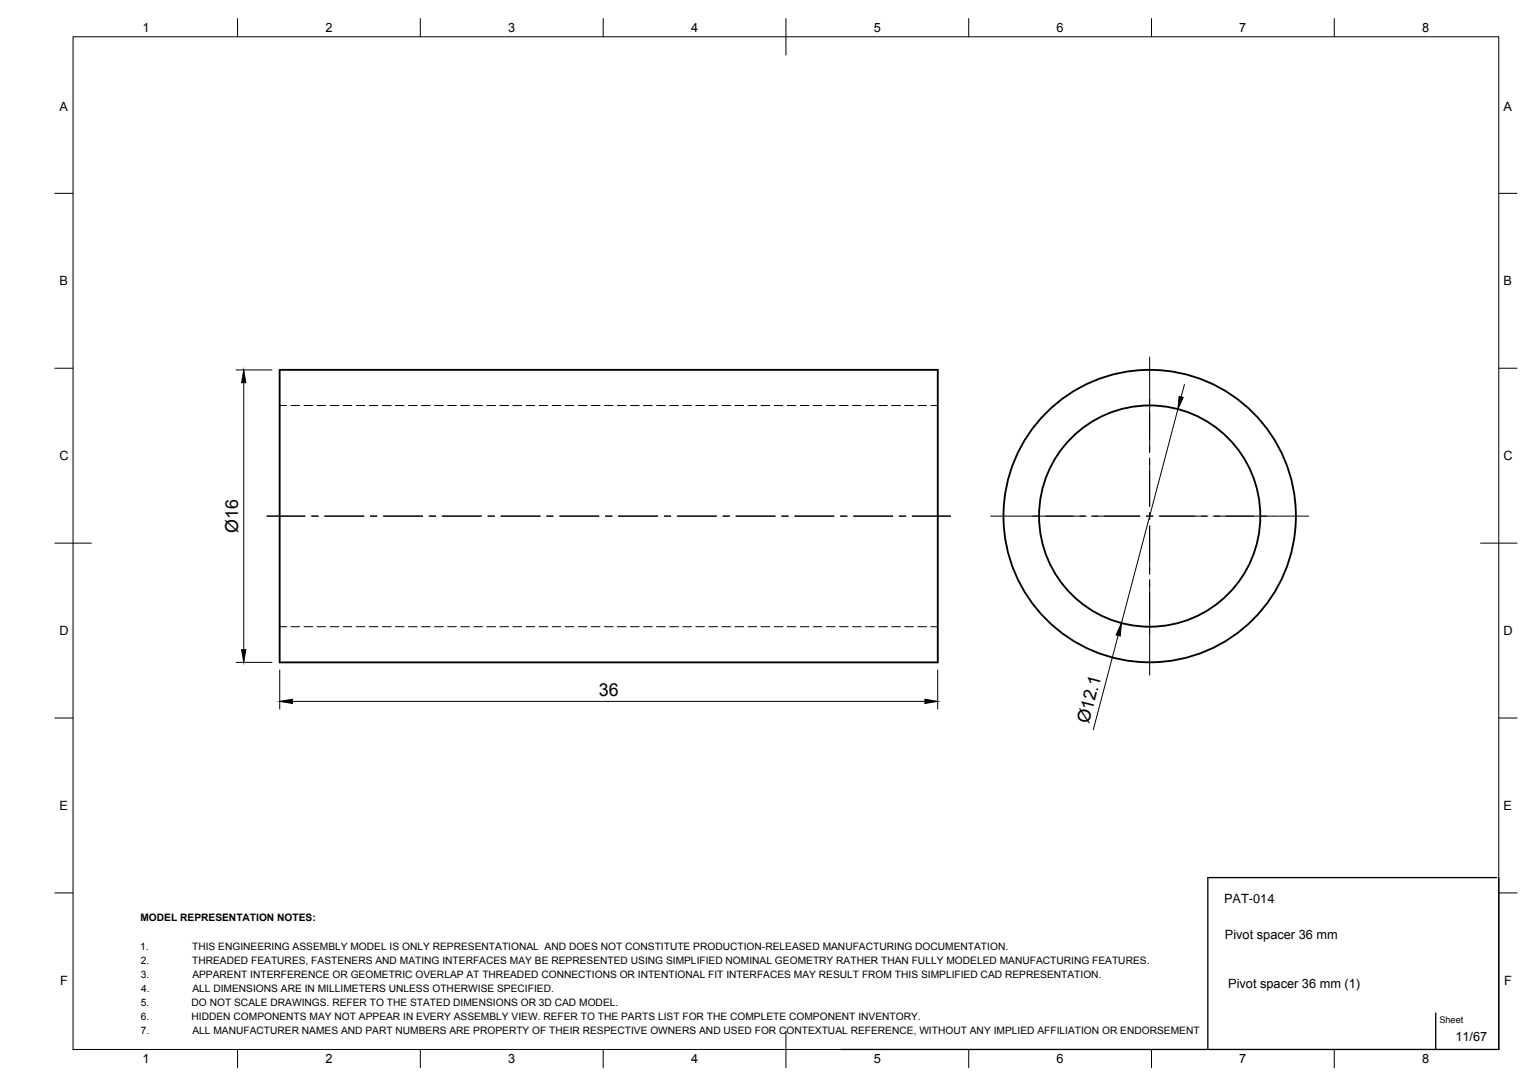
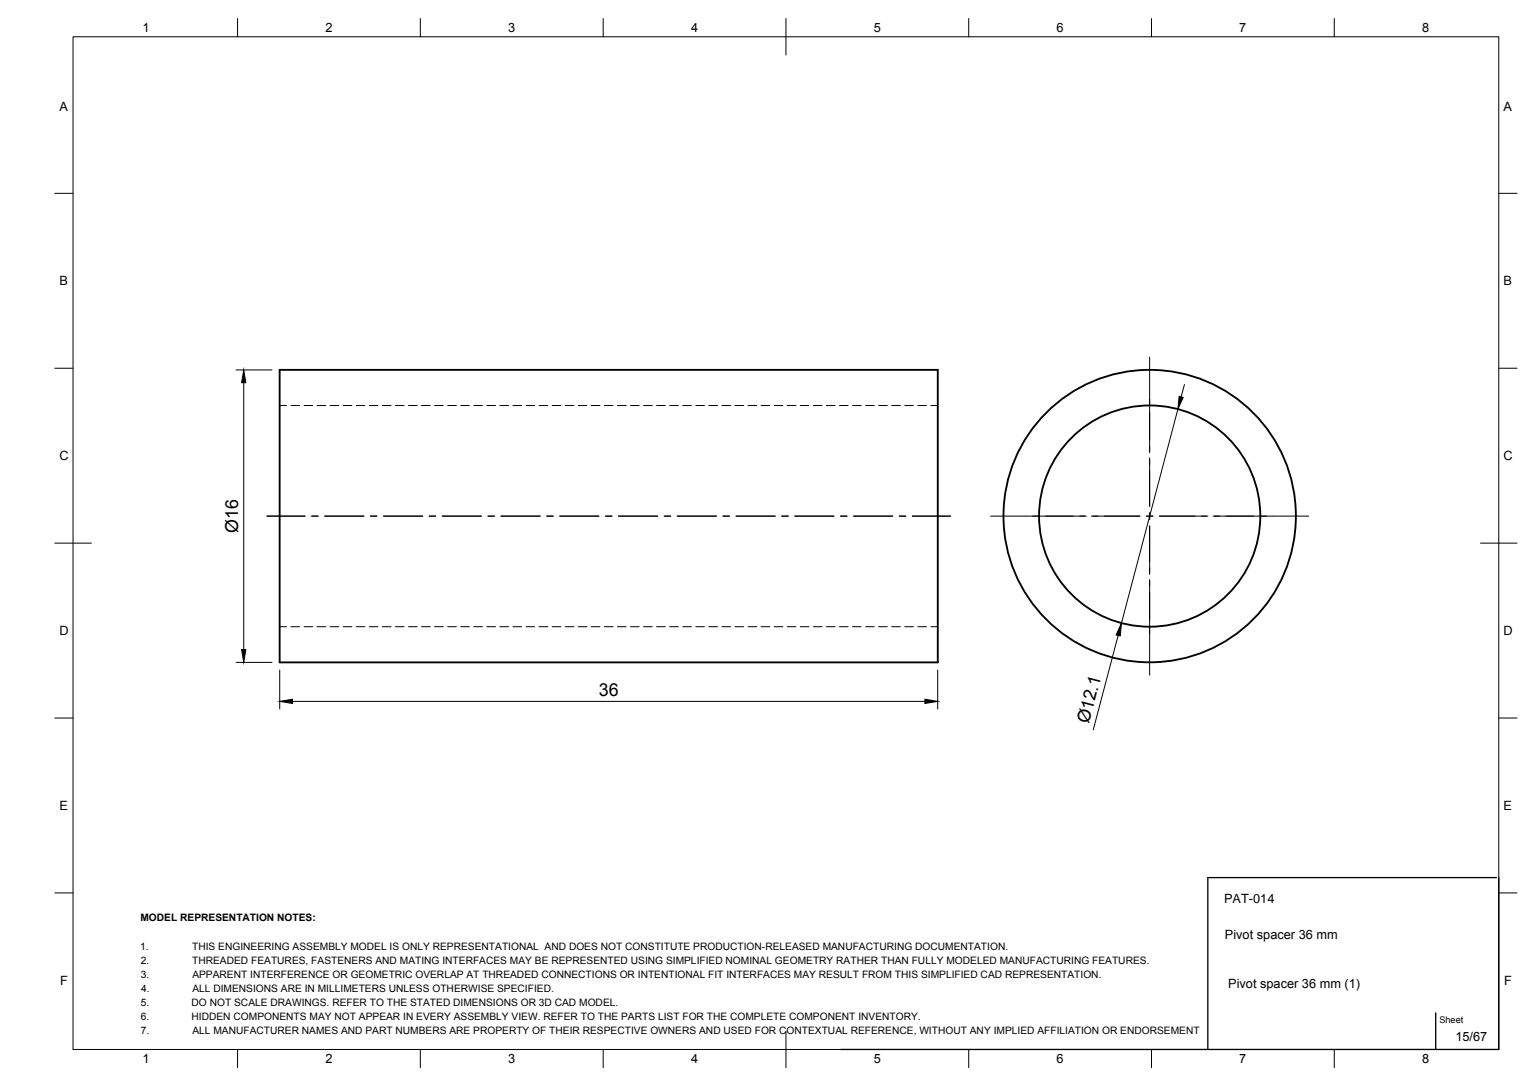
ISO-10303-21;
HEADER;
/* Generated by software containing ST-Developer
 * from STEP Tools, Inc. (www.steptools.com) 
 */

FILE_DESCRIPTION(
/* description */ ('Bin tilter linkage'),
/* implementation_level */ '2;1');

FILE_NAME(
/* name */ 'Pivot spacer 36 mm (1).step',
/* time_stamp */ '2026-10-28T03:26:24-07:00',
/* author */ (''),
/* organization */ (''),
/* preprocessor_version */ 'ST-DEVELOPER v20.2',
/* originating_system */ 'Autodesk Translation Framework v15.17.0.0',
/* authorisation */ '');

FILE_SCHEMA (('AUTOMOTIVE_DESIGN { 1 0 10303 214 3 1 1 }'));
ENDSEC;

DATA;
#10=MECHANICAL_DESIGN_GEOMETRIC_PRESENTATION_REPRESENTATION('',(#872),#23728);
#660=SHAPE_REPRESENTATION_RELATIONSHIP('SRR','None',#24124,#766);
#766=ADVANCED_BREP_SHAPE_REPRESENTATION('',(#986),#23624);
#872=STYLED_ITEM('',(#24758),#986);
#986=MANIFOLD_SOLID_BREP('Body1',#12402);
#1167=FACE_BOUND('',#2852,.T.);
#1168=FACE_BOUND('',#2854,.T.);
#1546=PLANE('',#13893);
#1547=PLANE('',#13894);
#1992=FACE_OUTER_BOUND('',#2849,.T.);
#1993=FACE_OUTER_BOUND('',#2850,.T.);
#1994=FACE_OUTER_BOUND('',#2851,.T.);
#1995=FACE_OUTER_BOUND('',#2853,.T.);
#2849=EDGE_LOOP('',(#8829,#8830,#8831,#8832));
#2850=EDGE_LOOP('',(#8833,#8834,#8835,#8836));
#2851=EDGE_LOOP('',(#8837));
#2852=EDGE_LOOP('',(#8838));
#2853=EDGE_LOOP('',(#8839));
#2854=EDGE_LOOP('',(#8840));
#3981=LINE('',#20244,#4656);
#3982=LINE('',#20250,#4657);
#4656=VECTOR('',#16032,0.605);
#4657=VECTOR('',#16039,0.800000000000001);
#5295=CIRCLE('',#13888,0.605);
#5296=CIRCLE('',#13889,0.605);
#5297=CIRCLE('',#13891,0.800000000000001);
#5298=CIRCLE('',#13892,0.800000000000001);
#6109=VERTEX_POINT('',#20241);
#6110=VERTEX_POINT('',#20243);
#6111=VERTEX_POINT('',#20247);
#6112=VERTEX_POINT('',#20249);
#7154=EDGE_CURVE('',#6109,#6109,#5295,.T.);
#7155=EDGE_CURVE('',#6109,#6110,#3981,.T.);
#7156=EDGE_CURVE('',#6110,#6110,#5296,.T.);
#7157=EDGE_CURVE('',#6111,#6111,#5297,.T.);
#7158=EDGE_CURVE('',#6111,#6112,#3982,.T.);
#7159=EDGE_CURVE('',#6112,#6112,#5298,.T.);
#8829=ORIENTED_EDGE('',*,*,#7154,.F.);
#8830=ORIENTED_EDGE('',*,*,#7155,.T.);
#8831=ORIENTED_EDGE('',*,*,#7156,.T.);
#8832=ORIENTED_EDGE('',*,*,#7155,.F.);
#8833=ORIENTED_EDGE('',*,*,#7157,.F.);
#8834=ORIENTED_EDGE('',*,*,#7158,.T.);
#8835=ORIENTED_EDGE('',*,*,#7159,.T.);
#8836=ORIENTED_EDGE('',*,*,#7158,.F.);
#8837=ORIENTED_EDGE('',*,*,#7157,.T.);
#8838=ORIENTED_EDGE('',*,*,#7154,.T.);
#8839=ORIENTED_EDGE('',*,*,#7159,.F.);
#8840=ORIENTED_EDGE('',*,*,#7156,.F.);
#11315=CYLINDRICAL_SURFACE('',#13887,0.605);
#11316=CYLINDRICAL_SURFACE('',#13890,0.800000000000001);
#11717=ADVANCED_FACE('',(#1992),#11315,.F.);
#11718=ADVANCED_FACE('',(#1993),#11316,.T.);
#11719=ADVANCED_FACE('',(#1994,#1167),#1546,.T.);
#11720=ADVANCED_FACE('',(#1995,#1168),#1547,.F.);
#12402=CLOSED_SHELL('',(#11717,#11718,#11719,#11720));
#13886=AXIS2_PLACEMENT_3D('',#20239,#16026,#16027);
#13887=AXIS2_PLACEMENT_3D('',#20240,#16028,#16029);
#13888=AXIS2_PLACEMENT_3D('',#20242,#16030,#16031);
#13889=AXIS2_PLACEMENT_3D('',#20245,#16033,#16034);
#13890=AXIS2_PLACEMENT_3D('',#20246,#16035,#16036);
#13891=AXIS2_PLACEMENT_3D('',#20248,#16037,#16038);
#13892=AXIS2_PLACEMENT_3D('',#20251,#16040,#16041);
#13893=AXIS2_PLACEMENT_3D('',#20252,#16042,#16043);
#13894=AXIS2_PLACEMENT_3D('',#20253,#16044,#16045);
#16026=DIRECTION('axis',(0.,0.,1.));
#16027=DIRECTION('refdir',(1.,0.,0.));
#16028=DIRECTION('center_axis',(0.,1.,0.));
#16029=DIRECTION('ref_axis',(1.,0.,0.));
#16030=DIRECTION('center_axis',(0.,-1.,0.));
#16031=DIRECTION('ref_axis',(1.,0.,0.));
#16032=DIRECTION('',(0.,-1.,0.));
#16033=DIRECTION('center_axis',(0.,-1.,0.));
#16034=DIRECTION('ref_axis',(1.,0.,0.));
#16035=DIRECTION('center_axis',(0.,1.,0.));
#16036=DIRECTION('ref_axis',(1.,0.,0.));
#16037=DIRECTION('center_axis',(0.,1.,0.));
#16038=DIRECTION('ref_axis',(1.,0.,0.));
#16039=DIRECTION('',(0.,-1.,0.));
#16040=DIRECTION('center_axis',(0.,1.,0.));
#16041=DIRECTION('ref_axis',(1.,0.,0.));
#16042=DIRECTION('center_axis',(0.,1.,0.));
#16043=DIRECTION('ref_axis',(1.,0.,0.));
#16044=DIRECTION('center_axis',(0.,1.,0.));
#16045=DIRECTION('ref_axis',(1.,0.,0.));
#20239=CARTESIAN_POINT('',(0.,0.,0.));
#20240=CARTESIAN_POINT('Origin',(18.,0.5,15.));
#20241=CARTESIAN_POINT('',(17.395,4.1,15.));
#20242=CARTESIAN_POINT('Origin',(18.,4.1,15.));
#20243=CARTESIAN_POINT('',(17.395,0.5,15.));
#20244=CARTESIAN_POINT('',(17.395,0.5,15.));
#20245=CARTESIAN_POINT('Origin',(18.,0.5,15.));
#20246=CARTESIAN_POINT('Origin',(18.,0.5,15.));
#20247=CARTESIAN_POINT('',(17.2,4.1,15.));
#20248=CARTESIAN_POINT('Origin',(18.,4.1,15.));
#20249=CARTESIAN_POINT('',(17.2,0.5,15.));
#20250=CARTESIAN_POINT('',(17.2,0.5,15.));
#20251=CARTESIAN_POINT('Origin',(18.,0.5,15.));
#20252=CARTESIAN_POINT('Origin',(18.,4.1,15.));
#20253=CARTESIAN_POINT('Origin',(18.,0.5,15.));
#23507=UNCERTAINTY_MEASURE_WITH_UNIT(LENGTH_MEASURE(0.001),#23729,
'DISTANCE_ACCURACY_VALUE',
'Maximum model space distance between geometric entities at asserted c
onnectivities');
#23611=UNCERTAINTY_MEASURE_WITH_UNIT(LENGTH_MEASURE(0.001),#23729,
'DISTANCE_ACCURACY_VALUE',
'Maximum model space distance between geometric entities at asserted c
onnectivities');
#23624=(
GEOMETRIC_REPRESENTATION_CONTEXT(3)
GLOBAL_UNCERTAINTY_ASSIGNED_CONTEXT((#23507))
GLOBAL_UNIT_ASSIGNED_CONTEXT((#23729,#23731,#23732))
REPRESENTATION_CONTEXT('','3D')
);
#23728=(
GEOMETRIC_REPRESENTATION_CONTEXT(3)
GLOBAL_UNCERTAINTY_ASSIGNED_CONTEXT((#23611))
GLOBAL_UNIT_ASSIGNED_CONTEXT((#23729,#23731,#23732))
REPRESENTATION_CONTEXT('','3D')
);
#23729=(
LENGTH_UNIT()
NAMED_UNIT(*)
SI_UNIT(.CENTI.,.METRE.)
);
#23731=(
NAMED_UNIT(*)
PLANE_ANGLE_UNIT()
SI_UNIT($,.RADIAN.)
);
#23732=(
NAMED_UNIT(*)
SI_UNIT($,.STERADIAN.)
SOLID_ANGLE_UNIT()
);
#23745=SHAPE_DEFINITION_REPRESENTATION(#23861,#24124);
#23861=PRODUCT_DEFINITION_SHAPE('',$,#24241);
#24124=SHAPE_REPRESENTATION('',(#13886),#23624);
#24228=PRODUCT_DEFINITION_CONTEXT('part definition',#24578,'design');
#24241=PRODUCT_DEFINITION('Pivot spacer 36 mm (1)',
'Pivot spacer 36 mm (1)',#24357,#24228);
#24357=PRODUCT_DEFINITION_FORMATION('',$,#24592);
#24578=APPLICATION_CONTEXT(
'Core Data for Automotive Mechanical Design Process');
#24579=PRODUCT_CONTEXT('part definition',#24578,'mechanical');
#24592=PRODUCT('Pivot spacer 36 mm (1)','Pivot spacer 36 mm (1)',
'Pivot spacer 36 mm (1)',(#24579));
#24752=COLOUR_RGB('Sky Blue',0.24,0.69,0.87);
#24753=FILL_AREA_STYLE_COLOUR('',#24752);
#24754=FILL_AREA_STYLE('',(#24753));
#24755=SURFACE_STYLE_FILL_AREA(#24754);
#24756=SURFACE_SIDE_STYLE('',(#24755));
#24757=SURFACE_STYLE_USAGE(.BOTH.,#24756);
#24758=PRESENTATION_STYLE_ASSIGNMENT((#24757));
ENDSEC;
END-ISO-10303-21;
